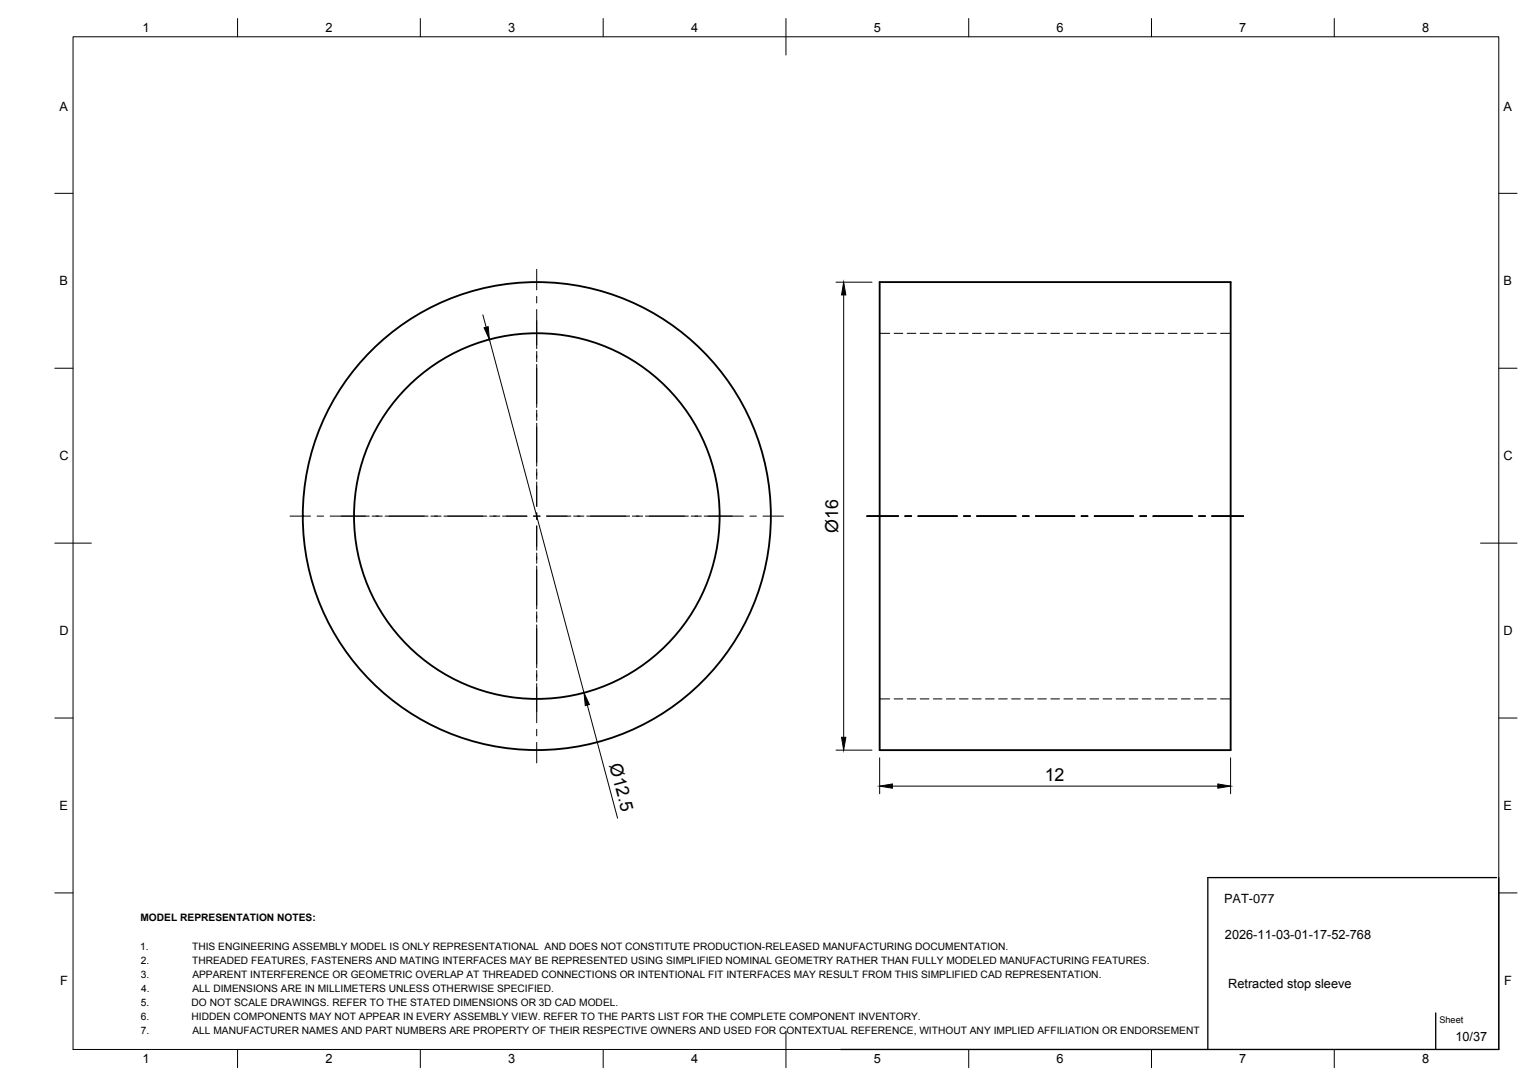
ISO-10303-21;
HEADER;
/* Generated by software containing ST-Developer
 * from STEP Tools, Inc. (www.steptools.com) 
 */

FILE_DESCRIPTION(
/* description */ ('Pallet stop with pneumatic fitting'),
/* implementation_level */ '2;1');

FILE_NAME(
/* name */ 'Retracted stop sleeve.step',
/* time_stamp */ '2026-10-27T10:51:41-07:00',
/* author */ (''),
/* organization */ (''),
/* preprocessor_version */ 'ST-DEVELOPER v20.2',
/* originating_system */ 'Autodesk Translation Framework v15.17.0.0',
/* authorisation */ '');

FILE_SCHEMA (('AUTOMOTIVE_DESIGN { 1 0 10303 214 3 1 1 }'));
ENDSEC;

DATA;
#10=MECHANICAL_DESIGN_GEOMETRIC_PRESENTATION_REPRESENTATION('',(#362),#10265);
#298=SHAPE_REPRESENTATION_RELATIONSHIP('SRR','None',#10411,#330);
#330=ADVANCED_BREP_SHAPE_REPRESENTATION('',(#394),#10235);
#362=STYLED_ITEM('',(#10648),#394);
#394=MANIFOLD_SOLID_BREP('Body1',#5050);
#463=FACE_BOUND('',#1167,.T.);
#464=FACE_BOUND('',#1169,.T.);
#585=PLANE('',#5576);
#586=PLANE('',#5577);
#806=FACE_OUTER_BOUND('',#1164,.T.);
#807=FACE_OUTER_BOUND('',#1165,.T.);
#808=FACE_OUTER_BOUND('',#1166,.T.);
#809=FACE_OUTER_BOUND('',#1168,.T.);
#1164=EDGE_LOOP('',(#3686,#3687,#3688,#3689));
#1165=EDGE_LOOP('',(#3690,#3691,#3692,#3693));
#1166=EDGE_LOOP('',(#3694));
#1167=EDGE_LOOP('',(#3695));
#1168=EDGE_LOOP('',(#3696));
#1169=EDGE_LOOP('',(#3697));
#1568=LINE('',#8050,#1903);
#1569=LINE('',#8056,#1904);
#1903=VECTOR('',#6447,0.625);
#1904=VECTOR('',#6454,0.8);
#2220=CIRCLE('',#5571,0.625);
#2221=CIRCLE('',#5572,0.625);
#2222=CIRCLE('',#5574,0.8);
#2223=CIRCLE('',#5575,0.8);
#2499=VERTEX_POINT('',#8047);
#2500=VERTEX_POINT('',#8049);
#2501=VERTEX_POINT('',#8053);
#2502=VERTEX_POINT('',#8055);
#2942=EDGE_CURVE('',#2499,#2499,#2220,.T.);
#2943=EDGE_CURVE('',#2499,#2500,#1568,.T.);
#2944=EDGE_CURVE('',#2500,#2500,#2221,.T.);
#2945=EDGE_CURVE('',#2501,#2501,#2222,.T.);
#2946=EDGE_CURVE('',#2501,#2502,#1569,.T.);
#2947=EDGE_CURVE('',#2502,#2502,#2223,.T.);
#3686=ORIENTED_EDGE('',*,*,#2942,.F.);
#3687=ORIENTED_EDGE('',*,*,#2943,.T.);
#3688=ORIENTED_EDGE('',*,*,#2944,.T.);
#3689=ORIENTED_EDGE('',*,*,#2943,.F.);
#3690=ORIENTED_EDGE('',*,*,#2945,.F.);
#3691=ORIENTED_EDGE('',*,*,#2946,.T.);
#3692=ORIENTED_EDGE('',*,*,#2947,.T.);
#3693=ORIENTED_EDGE('',*,*,#2946,.F.);
#3694=ORIENTED_EDGE('',*,*,#2945,.T.);
#3695=ORIENTED_EDGE('',*,*,#2942,.T.);
#3696=ORIENTED_EDGE('',*,*,#2947,.F.);
#3697=ORIENTED_EDGE('',*,*,#2944,.F.);
#4652=CYLINDRICAL_SURFACE('',#5570,0.625);
#4653=CYLINDRICAL_SURFACE('',#5573,0.8);
#4801=ADVANCED_FACE('',(#806),#4652,.F.);
#4802=ADVANCED_FACE('',(#807),#4653,.T.);
#4803=ADVANCED_FACE('',(#808,#463),#585,.T.);
#4804=ADVANCED_FACE('',(#809,#464),#586,.F.);
#5050=CLOSED_SHELL('',(#4801,#4802,#4803,#4804));
#5569=AXIS2_PLACEMENT_3D('',#8045,#6441,#6442);
#5570=AXIS2_PLACEMENT_3D('',#8046,#6443,#6444);
#5571=AXIS2_PLACEMENT_3D('',#8048,#6445,#6446);
#5572=AXIS2_PLACEMENT_3D('',#8051,#6448,#6449);
#5573=AXIS2_PLACEMENT_3D('',#8052,#6450,#6451);
#5574=AXIS2_PLACEMENT_3D('',#8054,#6452,#6453);
#5575=AXIS2_PLACEMENT_3D('',#8057,#6455,#6456);
#5576=AXIS2_PLACEMENT_3D('',#8058,#6457,#6458);
#5577=AXIS2_PLACEMENT_3D('',#8059,#6459,#6460);
#6441=DIRECTION('axis',(0.,0.,1.));
#6442=DIRECTION('refdir',(1.,0.,0.));
#6443=DIRECTION('center_axis',(0.,0.,1.));
#6444=DIRECTION('ref_axis',(1.,0.,0.));
#6445=DIRECTION('center_axis',(0.,0.,-1.));
#6446=DIRECTION('ref_axis',(1.,0.,0.));
#6447=DIRECTION('',(0.,0.,-1.));
#6448=DIRECTION('center_axis',(0.,0.,-1.));
#6449=DIRECTION('ref_axis',(1.,0.,0.));
#6450=DIRECTION('center_axis',(0.,0.,1.));
#6451=DIRECTION('ref_axis',(1.,0.,0.));
#6452=DIRECTION('center_axis',(0.,0.,1.));
#6453=DIRECTION('ref_axis',(1.,0.,0.));
#6454=DIRECTION('',(0.,0.,-1.));
#6455=DIRECTION('center_axis',(0.,0.,1.));
#6456=DIRECTION('ref_axis',(1.,0.,0.));
#6457=DIRECTION('center_axis',(0.,0.,1.));
#6458=DIRECTION('ref_axis',(1.,0.,0.));
#6459=DIRECTION('center_axis',(0.,0.,1.));
#6460=DIRECTION('ref_axis',(1.,0.,0.));
#8045=CARTESIAN_POINT('',(0.,0.,0.));
#8046=CARTESIAN_POINT('Origin',(0.,0.,8.8));
#8047=CARTESIAN_POINT('',(-0.625,-7.65404249467096E-17,10.));
#8048=CARTESIAN_POINT('Origin',(0.,0.,10.));
#8049=CARTESIAN_POINT('',(-0.625,-7.65404249467096E-17,8.8));
#8050=CARTESIAN_POINT('',(-0.625,-7.65404249467096E-17,8.8));
#8051=CARTESIAN_POINT('Origin',(0.,0.,8.8));
#8052=CARTESIAN_POINT('Origin',(0.,0.,8.8));
#8053=CARTESIAN_POINT('',(-0.8,-9.79717439317883E-17,10.));
#8054=CARTESIAN_POINT('Origin',(0.,0.,10.));
#8055=CARTESIAN_POINT('',(-0.8,-9.79717439317883E-17,8.8));
#8056=CARTESIAN_POINT('',(-0.8,-9.79717439317883E-17,8.8));
#8057=CARTESIAN_POINT('Origin',(0.,0.,8.8));
#8058=CARTESIAN_POINT('Origin',(0.,0.,10.));
#8059=CARTESIAN_POINT('Origin',(0.,0.,8.8));
#10197=UNCERTAINTY_MEASURE_WITH_UNIT(LENGTH_MEASURE(0.001),#10266,
'DISTANCE_ACCURACY_VALUE',
'Maximum model space distance between geometric entities at asserted c
onnectivities');
#10227=UNCERTAINTY_MEASURE_WITH_UNIT(LENGTH_MEASURE(0.001),#10266,
'DISTANCE_ACCURACY_VALUE',
'Maximum model space distance between geometric entities at asserted c
onnectivities');
#10235=(
GEOMETRIC_REPRESENTATION_CONTEXT(3)
GLOBAL_UNCERTAINTY_ASSIGNED_CONTEXT((#10197))
GLOBAL_UNIT_ASSIGNED_CONTEXT((#10266,#10268,#10269))
REPRESENTATION_CONTEXT('','3D')
);
#10265=(
GEOMETRIC_REPRESENTATION_CONTEXT(3)
GLOBAL_UNCERTAINTY_ASSIGNED_CONTEXT((#10227))
GLOBAL_UNIT_ASSIGNED_CONTEXT((#10266,#10268,#10269))
REPRESENTATION_CONTEXT('','3D')
);
#10266=(
LENGTH_UNIT()
NAMED_UNIT(*)
SI_UNIT(.CENTI.,.METRE.)
);
#10268=(
NAMED_UNIT(*)
PLANE_ANGLE_UNIT()
SI_UNIT($,.RADIAN.)
);
#10269=(
NAMED_UNIT(*)
SI_UNIT($,.STERADIAN.)
SOLID_ANGLE_UNIT()
);
#10277=SHAPE_DEFINITION_REPRESENTATION(#10314,#10411);
#10314=PRODUCT_DEFINITION_SHAPE('',$,#10449);
#10411=SHAPE_REPRESENTATION('',(#5569),#10235);
#10441=PRODUCT_DEFINITION_CONTEXT('part definition',#10554,'design');
#10449=PRODUCT_DEFINITION('Retracted stop sleeve',
'Retracted stop sleeve',#10486,#10441);
#10486=PRODUCT_DEFINITION_FORMATION('',$,#10563);
#10554=APPLICATION_CONTEXT(
'Core Data for Automotive Mechanical Design Process');
#10555=PRODUCT_CONTEXT('part definition',#10554,'mechanical');
#10563=PRODUCT('Retracted stop sleeve','Retracted stop sleeve',
'Retracted stop sleeve',(#10555));
#10642=COLOUR_RGB('Sky Blue',0.24,0.69,0.87);
#10643=FILL_AREA_STYLE_COLOUR('',#10642);
#10644=FILL_AREA_STYLE('',(#10643));
#10645=SURFACE_STYLE_FILL_AREA(#10644);
#10646=SURFACE_SIDE_STYLE('',(#10645));
#10647=SURFACE_STYLE_USAGE(.BOTH.,#10646);
#10648=PRESENTATION_STYLE_ASSIGNMENT((#10647));
ENDSEC;
END-ISO-10303-21;
